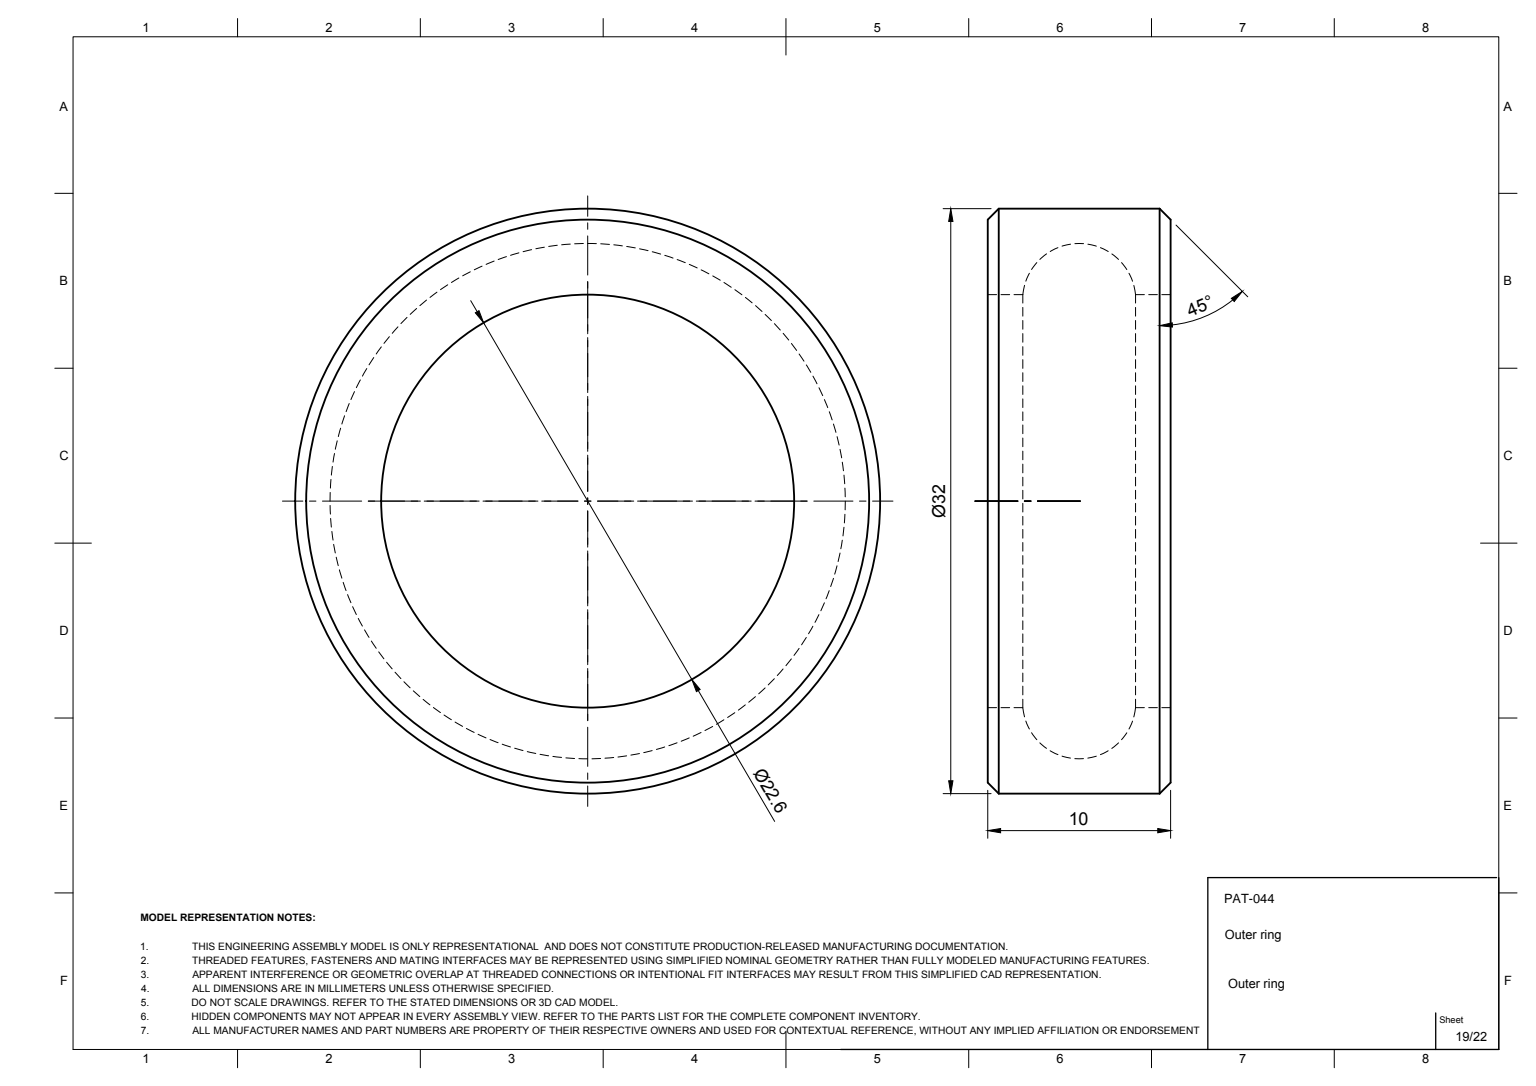
ISO-10303-21;
HEADER;
/* Generated by software containing ST-Developer
 * from STEP Tools, Inc. (www.steptools.com) 
 */

FILE_DESCRIPTION(
/* description */ ('Four-wheel beam trolley'),
/* implementation_level */ '2;1');

FILE_NAME(
/* name */ 'Outer ring.step',
/* time_stamp */ '2026-10-29T16:22:06-07:00',
/* author */ (''),
/* organization */ (''),
/* preprocessor_version */ 'ST-DEVELOPER v20.2',
/* originating_system */ 'Autodesk Translation Framework v15.17.0.0',
/* authorisation */ '');

FILE_SCHEMA (('AUTOMOTIVE_DESIGN { 1 0 10303 214 3 1 1 }'));
ENDSEC;

DATA;
#10=MECHANICAL_DESIGN_GEOMETRIC_PRESENTATION_REPRESENTATION('',(#290),#4777);
#40=TOROIDAL_SURFACE('',#2807,1.1,0.309556);
#240=CONICAL_SURFACE('',#2818,1.57,0.785398163397449);
#241=CONICAL_SURFACE('',#2822,1.57,0.785398163397449);
#256=SHAPE_REPRESENTATION_RELATIONSHIP('SRR','None',#4887,#273);
#273=ADVANCED_BREP_SHAPE_REPRESENTATION('',(#312),#4772);
#290=STYLED_ITEM('',(#5056),#312);
#312=MANIFOLD_SOLID_BREP('Body1',#2379);
#356=FACE_BOUND('',#727,.T.);
#357=FACE_BOUND('',#732,.T.);
#426=PLANE('',#2815);
#427=PLANE('',#2824);
#545=FACE_OUTER_BOUND('',#724,.T.);
#546=FACE_OUTER_BOUND('',#725,.T.);
#547=FACE_OUTER_BOUND('',#726,.T.);
#548=FACE_OUTER_BOUND('',#728,.T.);
#549=FACE_OUTER_BOUND('',#729,.T.);
#550=FACE_OUTER_BOUND('',#730,.T.);
#551=FACE_OUTER_BOUND('',#731,.T.);
#552=FACE_OUTER_BOUND('',#733,.T.);
#724=EDGE_LOOP('',(#1997,#1998,#1999,#2000,#2001,#2002));
#725=EDGE_LOOP('',(#2003,#2004,#2005,#2006,#2007));
#726=EDGE_LOOP('',(#2008));
#727=EDGE_LOOP('',(#2009));
#728=EDGE_LOOP('',(#2010,#2011,#2012,#2013));
#729=EDGE_LOOP('',(#2014,#2015,#2016,#2017));
#730=EDGE_LOOP('',(#2018,#2019,#2020,#2021));
#731=EDGE_LOOP('',(#2022));
#732=EDGE_LOOP('',(#2023));
#733=EDGE_LOOP('',(#2024,#2025,#2026,#2027,#2028));
#887=LINE('',#4233,#1010);
#888=LINE('',#4242,#1011);
#889=LINE('',#4246,#1012);
#890=LINE('',#4250,#1013);
#891=LINE('',#4253,#1014);
#1010=VECTOR('',#3514,1.129765);
#1011=VECTOR('',#3525,1.57);
#1012=VECTOR('',#3530,1.6);
#1013=VECTOR('',#3535,1.57);
#1014=VECTOR('',#3540,1.129765);
#1099=CIRCLE('',#2808,1.129765);
#1100=CIRCLE('',#2809,1.129765);
#1101=CIRCLE('',#2810,0.309556);
#1102=CIRCLE('',#2811,1.129765);
#1103=CIRCLE('',#2812,1.129765);
#1104=CIRCLE('',#2814,1.129765);
#1105=CIRCLE('',#2816,1.54);
#1106=CIRCLE('',#2817,1.129765);
#1107=CIRCLE('',#2819,1.6);
#1108=CIRCLE('',#2821,1.6);
#1109=CIRCLE('',#2823,1.54);
#1282=VERTEX_POINT('',#4221);
#1283=VERTEX_POINT('',#4222);
#1284=VERTEX_POINT('',#4225);
#1285=VERTEX_POINT('',#4227);
#1286=VERTEX_POINT('',#4231);
#1287=VERTEX_POINT('',#4235);
#1288=VERTEX_POINT('',#4237);
#1289=VERTEX_POINT('',#4240);
#1290=VERTEX_POINT('',#4244);
#1291=VERTEX_POINT('',#4248);
#1536=EDGE_CURVE('',#1282,#1283,#1099,.T.);
#1537=EDGE_CURVE('',#1283,#1282,#1100,.T.);
#1538=EDGE_CURVE('',#1283,#1284,#1101,.T.);
#1539=EDGE_CURVE('',#1285,#1284,#1102,.T.);
#1540=EDGE_CURVE('',#1284,#1285,#1103,.T.);
#1541=EDGE_CURVE('',#1286,#1286,#1104,.T.);
#1542=EDGE_CURVE('',#1286,#1285,#887,.T.);
#1543=EDGE_CURVE('',#1287,#1287,#1105,.T.);
#1544=EDGE_CURVE('',#1288,#1288,#1106,.T.);
#1545=EDGE_CURVE('',#1289,#1289,#1107,.T.);
#1546=EDGE_CURVE('',#1289,#1287,#888,.T.);
#1547=EDGE_CURVE('',#1290,#1290,#1108,.T.);
#1548=EDGE_CURVE('',#1290,#1289,#889,.T.);
#1549=EDGE_CURVE('',#1291,#1291,#1109,.T.);
#1550=EDGE_CURVE('',#1291,#1290,#890,.T.);
#1551=EDGE_CURVE('',#1282,#1288,#891,.T.);
#1997=ORIENTED_EDGE('',*,*,#1536,.F.);
#1998=ORIENTED_EDGE('',*,*,#1537,.F.);
#1999=ORIENTED_EDGE('',*,*,#1538,.T.);
#2000=ORIENTED_EDGE('',*,*,#1539,.F.);
#2001=ORIENTED_EDGE('',*,*,#1540,.F.);
#2002=ORIENTED_EDGE('',*,*,#1538,.F.);
#2003=ORIENTED_EDGE('',*,*,#1541,.T.);
#2004=ORIENTED_EDGE('',*,*,#1542,.T.);
#2005=ORIENTED_EDGE('',*,*,#1539,.T.);
#2006=ORIENTED_EDGE('',*,*,#1540,.T.);
#2007=ORIENTED_EDGE('',*,*,#1542,.F.);
#2008=ORIENTED_EDGE('',*,*,#1543,.F.);
#2009=ORIENTED_EDGE('',*,*,#1544,.T.);
#2010=ORIENTED_EDGE('',*,*,#1545,.F.);
#2011=ORIENTED_EDGE('',*,*,#1546,.T.);
#2012=ORIENTED_EDGE('',*,*,#1543,.T.);
#2013=ORIENTED_EDGE('',*,*,#1546,.F.);
#2014=ORIENTED_EDGE('',*,*,#1547,.F.);
#2015=ORIENTED_EDGE('',*,*,#1548,.T.);
#2016=ORIENTED_EDGE('',*,*,#1545,.T.);
#2017=ORIENTED_EDGE('',*,*,#1548,.F.);
#2018=ORIENTED_EDGE('',*,*,#1549,.F.);
#2019=ORIENTED_EDGE('',*,*,#1550,.T.);
#2020=ORIENTED_EDGE('',*,*,#1547,.T.);
#2021=ORIENTED_EDGE('',*,*,#1550,.F.);
#2022=ORIENTED_EDGE('',*,*,#1549,.T.);
#2023=ORIENTED_EDGE('',*,*,#1541,.F.);
#2024=ORIENTED_EDGE('',*,*,#1536,.T.);
#2025=ORIENTED_EDGE('',*,*,#1537,.T.);
#2026=ORIENTED_EDGE('',*,*,#1551,.T.);
#2027=ORIENTED_EDGE('',*,*,#1544,.F.);
#2028=ORIENTED_EDGE('',*,*,#1551,.F.);
#2207=CYLINDRICAL_SURFACE('',#2813,1.129765);
#2208=CYLINDRICAL_SURFACE('',#2820,1.6);
#2209=CYLINDRICAL_SURFACE('',#2825,1.129765);
#2321=ADVANCED_FACE('',(#545),#40,.F.);
#2322=ADVANCED_FACE('',(#546),#2207,.F.);
#2323=ADVANCED_FACE('',(#547,#356),#426,.T.);
#2324=ADVANCED_FACE('',(#548),#240,.T.);
#2325=ADVANCED_FACE('',(#549),#2208,.T.);
#2326=ADVANCED_FACE('',(#550),#241,.T.);
#2327=ADVANCED_FACE('',(#551,#357),#427,.T.);
#2328=ADVANCED_FACE('',(#552),#2209,.F.);
#2379=CLOSED_SHELL('',(#2321,#2322,#2323,#2324,#2325,#2326,#2327,#2328));
#2806=AXIS2_PLACEMENT_3D('',#4219,#3496,#3497);
#2807=AXIS2_PLACEMENT_3D('',#4220,#3498,#3499);
#2808=AXIS2_PLACEMENT_3D('',#4223,#3500,#3501);
#2809=AXIS2_PLACEMENT_3D('',#4224,#3502,#3503);
#2810=AXIS2_PLACEMENT_3D('',#4226,#3504,#3505);
#2811=AXIS2_PLACEMENT_3D('',#4228,#3506,#3507);
#2812=AXIS2_PLACEMENT_3D('',#4229,#3508,#3509);
#2813=AXIS2_PLACEMENT_3D('',#4230,#3510,#3511);
#2814=AXIS2_PLACEMENT_3D('',#4232,#3512,#3513);
#2815=AXIS2_PLACEMENT_3D('',#4234,#3515,#3516);
#2816=AXIS2_PLACEMENT_3D('',#4236,#3517,#3518);
#2817=AXIS2_PLACEMENT_3D('',#4238,#3519,#3520);
#2818=AXIS2_PLACEMENT_3D('',#4239,#3521,#3522);
#2819=AXIS2_PLACEMENT_3D('',#4241,#3523,#3524);
#2820=AXIS2_PLACEMENT_3D('',#4243,#3526,#3527);
#2821=AXIS2_PLACEMENT_3D('',#4245,#3528,#3529);
#2822=AXIS2_PLACEMENT_3D('',#4247,#3531,#3532);
#2823=AXIS2_PLACEMENT_3D('',#4249,#3533,#3534);
#2824=AXIS2_PLACEMENT_3D('',#4251,#3536,#3537);
#2825=AXIS2_PLACEMENT_3D('',#4252,#3538,#3539);
#3496=DIRECTION('axis',(0.,0.,1.));
#3497=DIRECTION('refdir',(1.,0.,0.));
#3498=DIRECTION('center_axis',(0.,-1.,0.));
#3499=DIRECTION('ref_axis',(0.,0.,-1.));
#3500=DIRECTION('center_axis',(0.,-1.,0.));
#3501=DIRECTION('ref_axis',(1.,0.,0.));
#3502=DIRECTION('center_axis',(0.,-1.,0.));
#3503=DIRECTION('ref_axis',(1.,0.,0.));
#3504=DIRECTION('center_axis',(1.,0.,1.22464679914735E-16));
#3505=DIRECTION('ref_axis',(-1.22464679914735E-16,0.,1.));
#3506=DIRECTION('center_axis',(0.,1.,0.));
#3507=DIRECTION('ref_axis',(1.,0.,0.));
#3508=DIRECTION('center_axis',(0.,1.,0.));
#3509=DIRECTION('ref_axis',(1.,0.,0.));
#3510=DIRECTION('center_axis',(0.,-1.,0.));
#3511=DIRECTION('ref_axis',(1.,0.,0.));
#3512=DIRECTION('center_axis',(0.,-1.,0.));
#3513=DIRECTION('ref_axis',(1.,0.,0.));
#3514=DIRECTION('',(0.,1.,0.));
#3515=DIRECTION('center_axis',(0.,1.,0.));
#3516=DIRECTION('ref_axis',(0.,0.,1.));
#3517=DIRECTION('center_axis',(0.,-1.,0.));
#3518=DIRECTION('ref_axis',(1.,0.,0.));
#3519=DIRECTION('center_axis',(0.,-1.,0.));
#3520=DIRECTION('ref_axis',(1.,0.,0.));
#3521=DIRECTION('center_axis',(0.,-1.,0.));
#3522=DIRECTION('ref_axis',(1.,0.,0.));
#3523=DIRECTION('center_axis',(0.,-1.,0.));
#3524=DIRECTION('ref_axis',(1.,0.,0.));
#3525=DIRECTION('',(0.707106781186548,0.707106781186547,8.65956056235494E-17));
#3526=DIRECTION('center_axis',(0.,-1.,0.));
#3527=DIRECTION('ref_axis',(1.,0.,0.));
#3528=DIRECTION('center_axis',(0.,-1.,0.));
#3529=DIRECTION('ref_axis',(1.,0.,0.));
#3530=DIRECTION('',(0.,1.,0.));
#3531=DIRECTION('center_axis',(0.,1.,0.));
#3532=DIRECTION('ref_axis',(1.,0.,0.));
#3533=DIRECTION('center_axis',(0.,-1.,0.));
#3534=DIRECTION('ref_axis',(1.,0.,0.));
#3535=DIRECTION('',(-0.707106781186548,0.707106781186547,-8.65956056235494E-17));
#3536=DIRECTION('center_axis',(0.,-1.,0.));
#3537=DIRECTION('ref_axis',(0.,0.,-1.));
#3538=DIRECTION('center_axis',(0.,-1.,0.));
#3539=DIRECTION('ref_axis',(1.,0.,0.));
#3540=DIRECTION('',(0.,1.,0.));
#4219=CARTESIAN_POINT('',(0.,0.,0.));
#4220=CARTESIAN_POINT('Origin',(0.,0.,0.));
#4221=CARTESIAN_POINT('',(-1.129765,0.308121667383195,-1.38356309103871E-16));
#4222=CARTESIAN_POINT('',(-1.38356309103871E-16,0.308121667383195,1.129765));
#4223=CARTESIAN_POINT('Origin',(0.,0.308121667383195,0.));
#4224=CARTESIAN_POINT('Origin',(0.,0.308121667383195,0.));
#4225=CARTESIAN_POINT('',(-1.38356309103871E-16,-0.308121667383195,1.129765));
#4226=CARTESIAN_POINT('Origin',(-1.34711147906209E-16,0.,1.1));
#4227=CARTESIAN_POINT('',(-1.129765,-0.308121667383195,1.38356309103871E-16));
#4228=CARTESIAN_POINT('Origin',(0.,-0.308121667383195,0.));
#4229=CARTESIAN_POINT('Origin',(0.,-0.308121667383195,0.));
#4230=CARTESIAN_POINT('Origin',(0.,0.,0.));
#4231=CARTESIAN_POINT('',(-1.129765,-0.5,-1.38356309103871E-16));
#4232=CARTESIAN_POINT('Origin',(0.,-0.5,0.));
#4233=CARTESIAN_POINT('',(-1.129765,0.,-1.38356309103871E-16));
#4234=CARTESIAN_POINT('Origin',(1.54,0.5,0.));
#4235=CARTESIAN_POINT('',(-1.54,0.5,-1.88595607068692E-16));
#4236=CARTESIAN_POINT('Origin',(0.,0.5,0.));
#4237=CARTESIAN_POINT('',(-1.129765,0.5,-1.38356309103871E-16));
#4238=CARTESIAN_POINT('Origin',(0.,0.5,0.));
#4239=CARTESIAN_POINT('Origin',(0.,0.47,0.));
#4240=CARTESIAN_POINT('',(-1.6,0.44,-1.95943487863577E-16));
#4241=CARTESIAN_POINT('Origin',(0.,0.44,0.));
#4242=CARTESIAN_POINT('',(-1.57,0.47,-1.92269547466134E-16));
#4243=CARTESIAN_POINT('Origin',(0.,0.,0.));
#4244=CARTESIAN_POINT('',(-1.6,-0.44,-1.95943487863577E-16));
#4245=CARTESIAN_POINT('Origin',(0.,-0.44,0.));
#4246=CARTESIAN_POINT('',(-1.6,0.,-1.95943487863577E-16));
#4247=CARTESIAN_POINT('Origin',(0.,-0.47,0.));
#4248=CARTESIAN_POINT('',(-1.54,-0.5,-1.88595607068692E-16));
#4249=CARTESIAN_POINT('Origin',(0.,-0.5,0.));
#4250=CARTESIAN_POINT('',(-1.57,-0.47,-1.92269547466134E-16));
#4251=CARTESIAN_POINT('Origin',(1.129765,-0.5,0.));
#4252=CARTESIAN_POINT('Origin',(0.,0.,0.));
#4253=CARTESIAN_POINT('',(-1.129765,0.,-1.38356309103871E-16));
#4750=UNCERTAINTY_MEASURE_WITH_UNIT(LENGTH_MEASURE(0.001),#4778,
'DISTANCE_ACCURACY_VALUE',
'Maximum model space distance between geometric entities at asserted c
onnectivities');
#4755=UNCERTAINTY_MEASURE_WITH_UNIT(LENGTH_MEASURE(0.001),#4778,
'DISTANCE_ACCURACY_VALUE',
'Maximum model space distance between geometric entities at asserted c
onnectivities');
#4772=(
GEOMETRIC_REPRESENTATION_CONTEXT(3)
GLOBAL_UNCERTAINTY_ASSIGNED_CONTEXT((#4750))
GLOBAL_UNIT_ASSIGNED_CONTEXT((#4778,#4780,#4781))
REPRESENTATION_CONTEXT('','3D')
);
#4777=(
GEOMETRIC_REPRESENTATION_CONTEXT(3)
GLOBAL_UNCERTAINTY_ASSIGNED_CONTEXT((#4755))
GLOBAL_UNIT_ASSIGNED_CONTEXT((#4778,#4780,#4781))
REPRESENTATION_CONTEXT('','3D')
);
#4778=(
LENGTH_UNIT()
NAMED_UNIT(*)
SI_UNIT(.CENTI.,.METRE.)
);
#4780=(
NAMED_UNIT(*)
PLANE_ANGLE_UNIT()
SI_UNIT($,.RADIAN.)
);
#4781=(
NAMED_UNIT(*)
SI_UNIT($,.STERADIAN.)
SOLID_ANGLE_UNIT()
);
#4798=SHAPE_DEFINITION_REPRESENTATION(#4851,#4887);
#4851=PRODUCT_DEFINITION_SHAPE('',$,#4909);
#4887=SHAPE_REPRESENTATION('',(#2806),#4772);
#4892=PRODUCT_DEFINITION_CONTEXT('part definition',#4957,'design');
#4909=PRODUCT_DEFINITION('Outer ring','Outer ring',#4930,#4892);
#4930=PRODUCT_DEFINITION_FORMATION('',$,#4975);
#4957=APPLICATION_CONTEXT(
'Core Data for Automotive Mechanical Design Process');
#4958=PRODUCT_CONTEXT('part definition',#4957,'mechanical');
#4975=PRODUCT('Outer ring','Outer ring','Outer ring',(#4958));
#5050=COLOUR_RGB('Grey',0.48,0.52,0.57);
#5051=FILL_AREA_STYLE_COLOUR('',#5050);
#5052=FILL_AREA_STYLE('',(#5051));
#5053=SURFACE_STYLE_FILL_AREA(#5052);
#5054=SURFACE_SIDE_STYLE('',(#5053));
#5055=SURFACE_STYLE_USAGE(.BOTH.,#5054);
#5056=PRESENTATION_STYLE_ASSIGNMENT((#5055));
ENDSEC;
END-ISO-10303-21;
